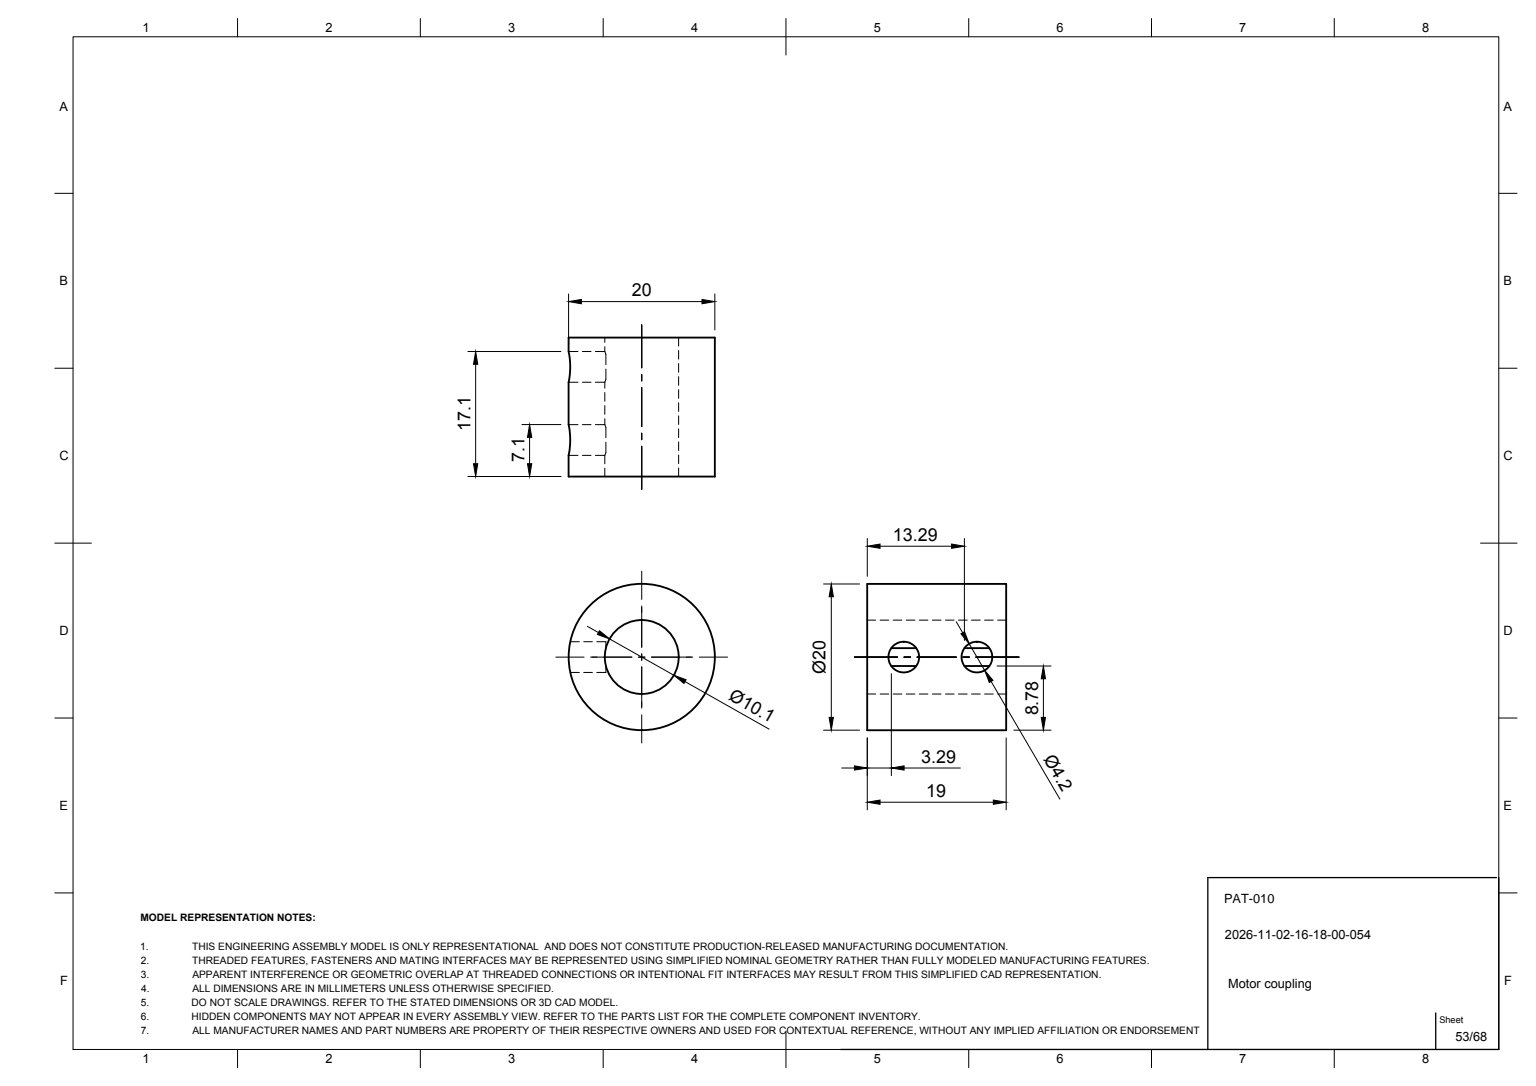
ISO-10303-21;
HEADER;
/* Generated by software containing ST-Developer
 * from STEP Tools, Inc. (www.steptools.com) 
 */

FILE_DESCRIPTION(
/* description */ ('Belt conveyor head drive unit'),
/* implementation_level */ '2;1');

FILE_NAME(
/* name */ 'Motor coupling.step',
/* time_stamp */ '2026-10-28T03:26:19-07:00',
/* author */ (''),
/* organization */ (''),
/* preprocessor_version */ 'ST-DEVELOPER v20.2',
/* originating_system */ 'Autodesk Translation Framework v15.17.0.0',
/* authorisation */ '');

FILE_SCHEMA (('AUTOMOTIVE_DESIGN { 1 0 10303 214 3 1 1 }'));
ENDSEC;

DATA;
#10=MECHANICAL_DESIGN_GEOMETRIC_PRESENTATION_REPRESENTATION('',(#914),#27069);
#577=B_SPLINE_CURVE_WITH_KNOTS('',3,(#24565,#24566,#24567,#24568,#24569,
#24570,#24571,#24572,#24573,#24574),.UNSPECIFIED.,.F.,.F.,(4,2,2,2,4),(0.83629428206811,
0.881958251377254,0.962083854030852,1.04220945668445,1.08787342599359),
 .UNSPECIFIED.);
#578=B_SPLINE_CURVE_WITH_KNOTS('',3,(#24580,#24581,#24582,#24583,#24584,
#24585,#24586,#24587,#24588,#24589,#24590,#24591,#24592,#24593,#24594,#24595,
#24596,#24597),.UNSPECIFIED.,.F.,.F.,(4,2,2,2,2,2,2,2,4),(0.,0.0793616477694785,
0.158723295538957,0.238079516586307,0.317435737633656,0.396791958681006,
0.476148179728355,0.555509827497834,0.634871475267312),.UNSPECIFIED.);
#579=B_SPLINE_CURVE_WITH_KNOTS('',3,(#24598,#24599,#24600,#24601,#24602,
#24603,#24604,#24605,#24606,#24607,#24608,#24609,#24610,#24611,#24612,#24613,
#24614,#24615),.UNSPECIFIED.,.F.,.F.,(4,2,2,2,2,2,2,2,4),(0.634871475267312,
0.714233123036791,0.793594770806269,0.872950991853619,0.952307212900968,
1.03166343394832,1.11101965499567,1.19038130276515,1.26974295053462),
 .UNSPECIFIED.);
#580=B_SPLINE_CURVE_WITH_KNOTS('',3,(#24618,#24619,#24620,#24621,#24622,
#24623,#24624,#24625,#24626,#24627),.UNSPECIFIED.,.F.,.F.,(4,2,2,2,4),(0.194905046047542,
0.240569015356686,0.320694618010284,0.400820220663882,0.446484189973025),
 .UNSPECIFIED.);
#581=B_SPLINE_CURVE_WITH_KNOTS('',3,(#24637,#24638,#24639,#24640,#24641,
#24642,#24643,#24644,#24645,#24646),.UNSPECIFIED.,.F.,.F.,(4,2,2,2,4),(0.83629428206811,
0.881958251377254,0.962083854030852,1.04220945668445,1.08787342599359),
 .UNSPECIFIED.);
#582=B_SPLINE_CURVE_WITH_KNOTS('',3,(#24652,#24653,#24654,#24655,#24656,
#24657,#24658,#24659,#24660,#24661,#24662,#24663,#24664,#24665,#24666,#24667,
#24668,#24669),.UNSPECIFIED.,.F.,.F.,(4,2,2,2,2,2,2,2,4),(0.,0.0793616477694785,
0.158723295538957,0.238079516586307,0.317435737633656,0.396791958681006,
0.476148179728355,0.555509827497834,0.634871475267312),.UNSPECIFIED.);
#583=B_SPLINE_CURVE_WITH_KNOTS('',3,(#24670,#24671,#24672,#24673,#24674,
#24675,#24676,#24677,#24678,#24679,#24680,#24681,#24682,#24683,#24684,#24685,
#24686,#24687),.UNSPECIFIED.,.F.,.F.,(4,2,2,2,2,2,2,2,4),(0.634871475267312,
0.714233123036791,0.793594770806269,0.872950991853619,0.952307212900968,
1.03166343394832,1.11101965499567,1.19038130276515,1.26974295053462),
 .UNSPECIFIED.);
#584=B_SPLINE_CURVE_WITH_KNOTS('',3,(#24690,#24691,#24692,#24693,#24694,
#24695,#24696,#24697,#24698,#24699),.UNSPECIFIED.,.F.,.F.,(4,2,2,2,4),(0.194905046047542,
0.240569015356686,0.320694618010284,0.400820220663882,0.446484189973025),
 .UNSPECIFIED.);
#760=SHAPE_REPRESENTATION_RELATIONSHIP('SRR','None',#27408,#829);
#829=ADVANCED_BREP_SHAPE_REPRESENTATION('',(#995),#27050);
#914=STYLED_ITEM('',(#27783),#995);
#995=MANIFOLD_SOLID_BREP('Body1',#13783);
#1216=FACE_BOUND('',#3192,.T.);
#1217=FACE_BOUND('',#3193,.T.);
#1218=FACE_BOUND('',#3195,.T.);
#1219=FACE_BOUND('',#3196,.T.);
#1220=FACE_BOUND('',#3198,.T.);
#1221=FACE_BOUND('',#3200,.T.);
#1560=PLANE('',#15709);
#1561=PLANE('',#15714);
#1562=PLANE('',#15715);
#1563=PLANE('',#15720);
#1564=PLANE('',#15727);
#1565=PLANE('',#15728);
#2181=FACE_OUTER_BOUND('',#3185,.T.);
#2182=FACE_OUTER_BOUND('',#3186,.T.);
#2183=FACE_OUTER_BOUND('',#3187,.T.);
#2184=FACE_OUTER_BOUND('',#3188,.T.);
#2185=FACE_OUTER_BOUND('',#3189,.T.);
#2186=FACE_OUTER_BOUND('',#3190,.T.);
#2187=FACE_OUTER_BOUND('',#3191,.T.);
#2188=FACE_OUTER_BOUND('',#3194,.T.);
#2189=FACE_OUTER_BOUND('',#3197,.T.);
#2190=FACE_OUTER_BOUND('',#3199,.T.);
#3185=EDGE_LOOP('',(#11250,#11251));
#3186=EDGE_LOOP('',(#11252,#11253,#11254,#11255,#11256,#11257,#11258,#11259,
#11260));
#3187=EDGE_LOOP('',(#11261,#11262,#11263));
#3188=EDGE_LOOP('',(#11264,#11265));
#3189=EDGE_LOOP('',(#11266,#11267,#11268,#11269,#11270,#11271,#11272,#11273,
#11274));
#3190=EDGE_LOOP('',(#11275,#11276,#11277));
#3191=EDGE_LOOP('',(#11278,#11279,#11280,#11281));
#3192=EDGE_LOOP('',(#11282,#11283,#11284,#11285));
#3193=EDGE_LOOP('',(#11286,#11287,#11288,#11289));
#3194=EDGE_LOOP('',(#11290,#11291,#11292,#11293));
#3195=EDGE_LOOP('',(#11294,#11295));
#3196=EDGE_LOOP('',(#11296,#11297));
#3197=EDGE_LOOP('',(#11298));
#3198=EDGE_LOOP('',(#11299));
#3199=EDGE_LOOP('',(#11300));
#3200=EDGE_LOOP('',(#11301));
#4059=LINE('',#24561,#4851);
#4060=LINE('',#24578,#4852);
#4061=LINE('',#24629,#4853);
#4062=LINE('',#24633,#4854);
#4063=LINE('',#24650,#4855);
#4064=LINE('',#24701,#4856);
#4065=LINE('',#24706,#4857);
#4066=LINE('',#24712,#4858);
#4851=VECTOR('',#19291,1.);
#4852=VECTOR('',#19298,0.21);
#4853=VECTOR('',#19303,1.);
#4854=VECTOR('',#19306,1.);
#4855=VECTOR('',#19313,0.21);
#4856=VECTOR('',#19318,1.);
#4857=VECTOR('',#19323,0.505);
#4858=VECTOR('',#19330,1.);
#5611=CIRCLE('',#15710,0.21);
#5612=CIRCLE('',#15712,0.21);
#5613=CIRCLE('',#15713,0.21);
#5614=CIRCLE('',#15716,0.21);
#5615=CIRCLE('',#15718,0.21);
#5616=CIRCLE('',#15719,0.21);
#5617=CIRCLE('',#15722,0.505);
#5618=CIRCLE('',#15723,0.505);
#5619=CIRCLE('',#15725,1.);
#5620=CIRCLE('',#15726,1.);
#6737=VERTEX_POINT('',#24559);
#6738=VERTEX_POINT('',#24560);
#6739=VERTEX_POINT('',#24564);
#6740=VERTEX_POINT('',#24575);
#6741=VERTEX_POINT('',#24577);
#6742=VERTEX_POINT('',#24579);
#6743=VERTEX_POINT('',#24616);
#6744=VERTEX_POINT('',#24631);
#6745=VERTEX_POINT('',#24632);
#6746=VERTEX_POINT('',#24636);
#6747=VERTEX_POINT('',#24647);
#6748=VERTEX_POINT('',#24649);
#6749=VERTEX_POINT('',#24651);
#6750=VERTEX_POINT('',#24688);
#6751=VERTEX_POINT('',#24703);
#6752=VERTEX_POINT('',#24705);
#6753=VERTEX_POINT('',#24709);
#6754=VERTEX_POINT('',#24711);
#8317=EDGE_CURVE('',#6737,#6738,#4059,.T.);
#8318=EDGE_CURVE('',#6737,#6738,#5611,.T.);
#8319=EDGE_CURVE('',#6739,#6737,#577,.T.);
#8320=EDGE_CURVE('',#6740,#6739,#5612,.T.);
#8321=EDGE_CURVE('',#6740,#6741,#4060,.T.);
#8322=EDGE_CURVE('',#6742,#6741,#578,.T.);
#8323=EDGE_CURVE('',#6741,#6742,#579,.T.);
#8324=EDGE_CURVE('',#6743,#6740,#5613,.T.);
#8325=EDGE_CURVE('',#6738,#6743,#580,.T.);
#8326=EDGE_CURVE('',#6743,#6739,#4061,.T.);
#8327=EDGE_CURVE('',#6744,#6745,#4062,.T.);
#8328=EDGE_CURVE('',#6744,#6745,#5614,.T.);
#8329=EDGE_CURVE('',#6746,#6744,#581,.T.);
#8330=EDGE_CURVE('',#6747,#6746,#5615,.T.);
#8331=EDGE_CURVE('',#6747,#6748,#4063,.T.);
#8332=EDGE_CURVE('',#6749,#6748,#582,.T.);
#8333=EDGE_CURVE('',#6748,#6749,#583,.T.);
#8334=EDGE_CURVE('',#6750,#6747,#5616,.T.);
#8335=EDGE_CURVE('',#6745,#6750,#584,.T.);
#8336=EDGE_CURVE('',#6750,#6746,#4064,.T.);
#8337=EDGE_CURVE('',#6751,#6751,#5617,.T.);
#8338=EDGE_CURVE('',#6751,#6752,#4065,.T.);
#8339=EDGE_CURVE('',#6752,#6752,#5618,.T.);
#8340=EDGE_CURVE('',#6753,#6753,#5619,.T.);
#8341=EDGE_CURVE('',#6753,#6754,#4066,.T.);
#8342=EDGE_CURVE('',#6754,#6754,#5620,.T.);
#11250=ORIENTED_EDGE('',*,*,#8317,.F.);
#11251=ORIENTED_EDGE('',*,*,#8318,.T.);
#11252=ORIENTED_EDGE('',*,*,#8319,.F.);
#11253=ORIENTED_EDGE('',*,*,#8320,.F.);
#11254=ORIENTED_EDGE('',*,*,#8321,.T.);
#11255=ORIENTED_EDGE('',*,*,#8322,.F.);
#11256=ORIENTED_EDGE('',*,*,#8323,.F.);
#11257=ORIENTED_EDGE('',*,*,#8321,.F.);
#11258=ORIENTED_EDGE('',*,*,#8324,.F.);
#11259=ORIENTED_EDGE('',*,*,#8325,.F.);
#11260=ORIENTED_EDGE('',*,*,#8318,.F.);
#11261=ORIENTED_EDGE('',*,*,#8326,.F.);
#11262=ORIENTED_EDGE('',*,*,#8324,.T.);
#11263=ORIENTED_EDGE('',*,*,#8320,.T.);
#11264=ORIENTED_EDGE('',*,*,#8327,.F.);
#11265=ORIENTED_EDGE('',*,*,#8328,.T.);
#11266=ORIENTED_EDGE('',*,*,#8329,.F.);
#11267=ORIENTED_EDGE('',*,*,#8330,.F.);
#11268=ORIENTED_EDGE('',*,*,#8331,.T.);
#11269=ORIENTED_EDGE('',*,*,#8332,.F.);
#11270=ORIENTED_EDGE('',*,*,#8333,.F.);
#11271=ORIENTED_EDGE('',*,*,#8331,.F.);
#11272=ORIENTED_EDGE('',*,*,#8334,.F.);
#11273=ORIENTED_EDGE('',*,*,#8335,.F.);
#11274=ORIENTED_EDGE('',*,*,#8328,.F.);
#11275=ORIENTED_EDGE('',*,*,#8336,.F.);
#11276=ORIENTED_EDGE('',*,*,#8334,.T.);
#11277=ORIENTED_EDGE('',*,*,#8330,.T.);
#11278=ORIENTED_EDGE('',*,*,#8337,.F.);
#11279=ORIENTED_EDGE('',*,*,#8338,.T.);
#11280=ORIENTED_EDGE('',*,*,#8339,.T.);
#11281=ORIENTED_EDGE('',*,*,#8338,.F.);
#11282=ORIENTED_EDGE('',*,*,#8325,.T.);
#11283=ORIENTED_EDGE('',*,*,#8326,.T.);
#11284=ORIENTED_EDGE('',*,*,#8319,.T.);
#11285=ORIENTED_EDGE('',*,*,#8317,.T.);
#11286=ORIENTED_EDGE('',*,*,#8335,.T.);
#11287=ORIENTED_EDGE('',*,*,#8336,.T.);
#11288=ORIENTED_EDGE('',*,*,#8329,.T.);
#11289=ORIENTED_EDGE('',*,*,#8327,.T.);
#11290=ORIENTED_EDGE('',*,*,#8340,.F.);
#11291=ORIENTED_EDGE('',*,*,#8341,.T.);
#11292=ORIENTED_EDGE('',*,*,#8342,.T.);
#11293=ORIENTED_EDGE('',*,*,#8341,.F.);
#11294=ORIENTED_EDGE('',*,*,#8322,.T.);
#11295=ORIENTED_EDGE('',*,*,#8323,.T.);
#11296=ORIENTED_EDGE('',*,*,#8332,.T.);
#11297=ORIENTED_EDGE('',*,*,#8333,.T.);
#11298=ORIENTED_EDGE('',*,*,#8340,.T.);
#11299=ORIENTED_EDGE('',*,*,#8337,.T.);
#11300=ORIENTED_EDGE('',*,*,#8342,.F.);
#11301=ORIENTED_EDGE('',*,*,#8339,.F.);
#12739=CYLINDRICAL_SURFACE('',#15711,0.21);
#12740=CYLINDRICAL_SURFACE('',#15717,0.21);
#12741=CYLINDRICAL_SURFACE('',#15721,0.505);
#12742=CYLINDRICAL_SURFACE('',#15724,1.);
#13460=ADVANCED_FACE('',(#2181),#1560,.T.);
#13461=ADVANCED_FACE('',(#2182),#12739,.F.);
#13462=ADVANCED_FACE('',(#2183),#1561,.T.);
#13463=ADVANCED_FACE('',(#2184),#1562,.T.);
#13464=ADVANCED_FACE('',(#2185),#12740,.F.);
#13465=ADVANCED_FACE('',(#2186),#1563,.T.);
#13466=ADVANCED_FACE('',(#2187,#1216,#1217),#12741,.F.);
#13467=ADVANCED_FACE('',(#2188,#1218,#1219),#12742,.T.);
#13468=ADVANCED_FACE('',(#2189,#1220),#1564,.T.);
#13469=ADVANCED_FACE('',(#2190,#1221),#1565,.F.);
#13783=CLOSED_SHELL('',(#13460,#13461,#13462,#13463,#13464,#13465,#13466,
#13467,#13468,#13469));
#15708=AXIS2_PLACEMENT_3D('',#24557,#19287,#19288);
#15709=AXIS2_PLACEMENT_3D('',#24558,#19289,#19290);
#15710=AXIS2_PLACEMENT_3D('',#24562,#19292,#19293);
#15711=AXIS2_PLACEMENT_3D('',#24563,#19294,#19295);
#15712=AXIS2_PLACEMENT_3D('',#24576,#19296,#19297);
#15713=AXIS2_PLACEMENT_3D('',#24617,#19299,#19300);
#15714=AXIS2_PLACEMENT_3D('',#24628,#19301,#19302);
#15715=AXIS2_PLACEMENT_3D('',#24630,#19304,#19305);
#15716=AXIS2_PLACEMENT_3D('',#24634,#19307,#19308);
#15717=AXIS2_PLACEMENT_3D('',#24635,#19309,#19310);
#15718=AXIS2_PLACEMENT_3D('',#24648,#19311,#19312);
#15719=AXIS2_PLACEMENT_3D('',#24689,#19314,#19315);
#15720=AXIS2_PLACEMENT_3D('',#24700,#19316,#19317);
#15721=AXIS2_PLACEMENT_3D('',#24702,#19319,#19320);
#15722=AXIS2_PLACEMENT_3D('',#24704,#19321,#19322);
#15723=AXIS2_PLACEMENT_3D('',#24707,#19324,#19325);
#15724=AXIS2_PLACEMENT_3D('',#24708,#19326,#19327);
#15725=AXIS2_PLACEMENT_3D('',#24710,#19328,#19329);
#15726=AXIS2_PLACEMENT_3D('',#24713,#19331,#19332);
#15727=AXIS2_PLACEMENT_3D('',#24714,#19333,#19334);
#15728=AXIS2_PLACEMENT_3D('',#24715,#19335,#19336);
#19287=DIRECTION('axis',(0.,0.,1.));
#19288=DIRECTION('refdir',(1.,0.,0.));
#19289=DIRECTION('center_axis',(0.,0.,1.));
#19290=DIRECTION('ref_axis',(1.,0.,0.));
#19291=DIRECTION('',(0.,1.,0.));
#19292=DIRECTION('center_axis',(0.,0.,1.));
#19293=DIRECTION('ref_axis',(1.,0.,0.));
#19294=DIRECTION('center_axis',(0.,0.,1.));
#19295=DIRECTION('ref_axis',(1.,0.,0.));
#19296=DIRECTION('center_axis',(0.,0.,1.));
#19297=DIRECTION('ref_axis',(1.,0.,0.));
#19298=DIRECTION('',(0.,0.,1.));
#19299=DIRECTION('center_axis',(0.,0.,1.));
#19300=DIRECTION('ref_axis',(1.,0.,0.));
#19301=DIRECTION('center_axis',(0.,0.,1.));
#19302=DIRECTION('ref_axis',(1.,0.,0.));
#19303=DIRECTION('',(0.,-1.,0.));
#19304=DIRECTION('center_axis',(0.,0.,1.));
#19305=DIRECTION('ref_axis',(1.,0.,0.));
#19306=DIRECTION('',(0.,1.,0.));
#19307=DIRECTION('center_axis',(0.,0.,1.));
#19308=DIRECTION('ref_axis',(1.,0.,0.));
#19309=DIRECTION('center_axis',(0.,0.,1.));
#19310=DIRECTION('ref_axis',(1.,0.,0.));
#19311=DIRECTION('center_axis',(0.,0.,1.));
#19312=DIRECTION('ref_axis',(1.,0.,0.));
#19313=DIRECTION('',(0.,0.,1.));
#19314=DIRECTION('center_axis',(0.,0.,1.));
#19315=DIRECTION('ref_axis',(1.,0.,0.));
#19316=DIRECTION('center_axis',(0.,0.,1.));
#19317=DIRECTION('ref_axis',(1.,0.,0.));
#19318=DIRECTION('',(0.,-1.,0.));
#19319=DIRECTION('center_axis',(0.,1.,0.));
#19320=DIRECTION('ref_axis',(1.,0.,0.));
#19321=DIRECTION('center_axis',(0.,-1.,0.));
#19322=DIRECTION('ref_axis',(1.,0.,0.));
#19323=DIRECTION('',(0.,-1.,0.));
#19324=DIRECTION('center_axis',(0.,-1.,0.));
#19325=DIRECTION('ref_axis',(1.,0.,0.));
#19326=DIRECTION('center_axis',(0.,1.,0.));
#19327=DIRECTION('ref_axis',(1.,0.,0.));
#19328=DIRECTION('center_axis',(0.,1.,0.));
#19329=DIRECTION('ref_axis',(1.,0.,0.));
#19330=DIRECTION('',(0.,-1.,0.));
#19331=DIRECTION('center_axis',(0.,1.,0.));
#19332=DIRECTION('ref_axis',(1.,0.,0.));
#19333=DIRECTION('center_axis',(0.,1.,0.));
#19334=DIRECTION('ref_axis',(1.,0.,0.));
#19335=DIRECTION('center_axis',(0.,1.,0.));
#19336=DIRECTION('ref_axis',(1.,0.,0.));
#24557=CARTESIAN_POINT('',(0.,0.,0.));
#24558=CARTESIAN_POINT('Origin',(0.,3.5,7.49));
#24559=CARTESIAN_POINT('',(0.122167917228702,3.32919309147461,7.49));
#24560=CARTESIAN_POINT('',(0.122167917228702,3.67080690852539,7.49));
#24561=CARTESIAN_POINT('',(0.122167917228702,2.1,7.49));
#24562=CARTESIAN_POINT('Origin',(0.,3.5,7.49));
#24563=CARTESIAN_POINT('Origin',(0.,3.5,7.49));
#24564=CARTESIAN_POINT('',(-0.122167917228702,3.32919309147461,7.49));
#24565=CARTESIAN_POINT('Ctrl Pts',(-0.122167917228702,3.32919309147461,
7.49));
#24566=CARTESIAN_POINT('Ctrl Pts',(-0.109498349122107,3.3201313107707,7.49315880560769));
#24567=CARTESIAN_POINT('Ctrl Pts',(-0.0955290239036627,3.31230742432584,
7.49610638003428));
#24568=CARTESIAN_POINT('Ctrl Pts',(-0.0549836006623198,3.29540341787373,
7.50267917175998));
#24569=CARTESIAN_POINT('Ctrl Pts',(-0.0267085342178658,3.29,7.505));
#24570=CARTESIAN_POINT('Ctrl Pts',(0.0267085342178659,3.29,7.505));
#24571=CARTESIAN_POINT('Ctrl Pts',(0.0549836006623198,3.29540341787373,
7.50267917175998));
#24572=CARTESIAN_POINT('Ctrl Pts',(0.0955290239036627,3.31230742432584,
7.49610638003428));
#24573=CARTESIAN_POINT('Ctrl Pts',(0.109498349122108,3.3201313107707,7.49315880560769));
#24574=CARTESIAN_POINT('Ctrl Pts',(0.122167917228702,3.32919309147461,7.49));
#24575=CARTESIAN_POINT('',(-0.21,3.5,7.49));
#24576=CARTESIAN_POINT('Origin',(0.,3.5,7.49));
#24577=CARTESIAN_POINT('',(-0.21,3.5,7.97770138590472));
#24578=CARTESIAN_POINT('',(-0.21,3.5,7.49));
#24579=CARTESIAN_POINT('',(0.21,3.5,7.97770138590472));
#24580=CARTESIAN_POINT('Ctrl Pts',(0.21,3.5,7.97770138590472));
#24581=CARTESIAN_POINT('Ctrl Pts',(0.21,3.47354611741017,7.97770138590472));
#24582=CARTESIAN_POINT('Ctrl Pts',(0.204697017125528,3.44538474169131,7.97888646613217));
#24583=CARTESIAN_POINT('Ctrl Pts',(0.183241751515529,3.39366957869826,7.98312869991148));
#24584=CARTESIAN_POINT('Ctrl Pts',(0.167093586802906,3.37010873870456,7.98612044796649));
#24585=CARTESIAN_POINT('Ctrl Pts',(0.129892533236543,3.33290768513819,7.99170645156379));
#24586=CARTESIAN_POINT('Ctrl Pts',(0.106331154992714,3.31675852489431,7.99466914446598));
#24587=CARTESIAN_POINT('Ctrl Pts',(0.0546141143983531,3.29530253627557,
7.99884449237241));
#24588=CARTESIAN_POINT('Ctrl Pts',(0.0264520736824499,3.29,8.));
#24589=CARTESIAN_POINT('Ctrl Pts',(-0.0264520736824498,3.29,8.));
#24590=CARTESIAN_POINT('Ctrl Pts',(-0.054614114398353,3.29530253627557,
7.99884449237241));
#24591=CARTESIAN_POINT('Ctrl Pts',(-0.106331154992714,3.31675852489431,
7.99466914446598));
#24592=CARTESIAN_POINT('Ctrl Pts',(-0.129892533236543,3.33290768513819,
7.99170645156379));
#24593=CARTESIAN_POINT('Ctrl Pts',(-0.167093586802906,3.37010873870456,
7.98612044796649));
#24594=CARTESIAN_POINT('Ctrl Pts',(-0.183241751515529,3.39366957869826,
7.98312869991148));
#24595=CARTESIAN_POINT('Ctrl Pts',(-0.204697017125528,3.44538474169131,
7.97888646613217));
#24596=CARTESIAN_POINT('Ctrl Pts',(-0.21,3.47354611741017,7.97770138590472));
#24597=CARTESIAN_POINT('Ctrl Pts',(-0.21,3.5,7.97770138590472));
#24598=CARTESIAN_POINT('Ctrl Pts',(-0.21,3.5,7.97770138590472));
#24599=CARTESIAN_POINT('Ctrl Pts',(-0.21,3.52645388258983,7.97770138590472));
#24600=CARTESIAN_POINT('Ctrl Pts',(-0.204697017125528,3.55461525830869,
7.97888646613217));
#24601=CARTESIAN_POINT('Ctrl Pts',(-0.183241751515529,3.60633042130174,
7.98312869991148));
#24602=CARTESIAN_POINT('Ctrl Pts',(-0.167093586802906,3.62989126129544,
7.98612044796649));
#24603=CARTESIAN_POINT('Ctrl Pts',(-0.129892533236543,3.66709231486181,
7.99170645156379));
#24604=CARTESIAN_POINT('Ctrl Pts',(-0.106331154992714,3.68324147510569,
7.99466914446598));
#24605=CARTESIAN_POINT('Ctrl Pts',(-0.0546141143983532,3.70469746372443,
7.99884449237241));
#24606=CARTESIAN_POINT('Ctrl Pts',(-0.0264520736824499,3.71,8.));
#24607=CARTESIAN_POINT('Ctrl Pts',(0.0264520736824498,3.71,8.));
#24608=CARTESIAN_POINT('Ctrl Pts',(0.0546141143983531,3.70469746372443,
7.99884449237241));
#24609=CARTESIAN_POINT('Ctrl Pts',(0.106331154992714,3.68324147510569,7.99466914446598));
#24610=CARTESIAN_POINT('Ctrl Pts',(0.129892533236543,3.66709231486181,7.99170645156379));
#24611=CARTESIAN_POINT('Ctrl Pts',(0.167093586802906,3.62989126129544,7.98612044796649));
#24612=CARTESIAN_POINT('Ctrl Pts',(0.183241751515529,3.60633042130174,7.98312869991148));
#24613=CARTESIAN_POINT('Ctrl Pts',(0.204697017125528,3.55461525830869,7.97888646613217));
#24614=CARTESIAN_POINT('Ctrl Pts',(0.21,3.52645388258983,7.97770138590472));
#24615=CARTESIAN_POINT('Ctrl Pts',(0.21,3.5,7.97770138590472));
#24616=CARTESIAN_POINT('',(-0.122167917228702,3.67080690852539,7.49));
#24617=CARTESIAN_POINT('Origin',(0.,3.5,7.49));
#24618=CARTESIAN_POINT('Ctrl Pts',(0.122167917228702,3.67080690852539,7.49));
#24619=CARTESIAN_POINT('Ctrl Pts',(0.109498349122108,3.6798686892293,7.49315880560769));
#24620=CARTESIAN_POINT('Ctrl Pts',(0.0955290239036627,3.68769257567416,
7.49610638003428));
#24621=CARTESIAN_POINT('Ctrl Pts',(0.0549836006623198,3.70459658212627,
7.50267917175998));
#24622=CARTESIAN_POINT('Ctrl Pts',(0.0267085342178658,3.71,7.505));
#24623=CARTESIAN_POINT('Ctrl Pts',(-0.0267085342178659,3.71,7.505));
#24624=CARTESIAN_POINT('Ctrl Pts',(-0.0549836006623198,3.70459658212627,
7.50267917175998));
#24625=CARTESIAN_POINT('Ctrl Pts',(-0.0955290239036627,3.68769257567416,
7.49610638003428));
#24626=CARTESIAN_POINT('Ctrl Pts',(-0.109498349122107,3.6798686892293,7.49315880560769));
#24627=CARTESIAN_POINT('Ctrl Pts',(-0.122167917228702,3.67080690852539,
7.49));
#24628=CARTESIAN_POINT('Origin',(0.,3.5,7.49));
#24629=CARTESIAN_POINT('',(-0.122167917228702,2.1,7.49));
#24630=CARTESIAN_POINT('Origin',(0.,2.5,7.49));
#24631=CARTESIAN_POINT('',(0.122167917228702,2.32919309147461,7.49));
#24632=CARTESIAN_POINT('',(0.122167917228702,2.67080690852539,7.49));
#24633=CARTESIAN_POINT('',(0.122167917228702,2.1,7.49));
#24634=CARTESIAN_POINT('Origin',(0.,2.5,7.49));
#24635=CARTESIAN_POINT('Origin',(0.,2.5,7.49));
#24636=CARTESIAN_POINT('',(-0.122167917228702,2.32919309147461,7.49));
#24637=CARTESIAN_POINT('Ctrl Pts',(-0.122167917228702,2.32919309147461,
7.49));
#24638=CARTESIAN_POINT('Ctrl Pts',(-0.109498349122107,2.3201313107707,7.49315880560769));
#24639=CARTESIAN_POINT('Ctrl Pts',(-0.0955290239036627,2.31230742432584,
7.49610638003428));
#24640=CARTESIAN_POINT('Ctrl Pts',(-0.0549836006623198,2.29540341787373,
7.50267917175998));
#24641=CARTESIAN_POINT('Ctrl Pts',(-0.0267085342178658,2.29,7.505));
#24642=CARTESIAN_POINT('Ctrl Pts',(0.0267085342178659,2.29,7.505));
#24643=CARTESIAN_POINT('Ctrl Pts',(0.0549836006623198,2.29540341787373,
7.50267917175998));
#24644=CARTESIAN_POINT('Ctrl Pts',(0.0955290239036627,2.31230742432584,
7.49610638003428));
#24645=CARTESIAN_POINT('Ctrl Pts',(0.109498349122107,2.3201313107707,7.49315880560769));
#24646=CARTESIAN_POINT('Ctrl Pts',(0.122167917228702,2.32919309147461,7.49));
#24647=CARTESIAN_POINT('',(-0.21,2.5,7.49));
#24648=CARTESIAN_POINT('Origin',(0.,2.5,7.49));
#24649=CARTESIAN_POINT('',(-0.21,2.5,7.97770138590472));
#24650=CARTESIAN_POINT('',(-0.21,2.5,7.49));
#24651=CARTESIAN_POINT('',(0.21,2.5,7.97770138590472));
#24652=CARTESIAN_POINT('Ctrl Pts',(0.21,2.5,7.97770138590472));
#24653=CARTESIAN_POINT('Ctrl Pts',(0.21,2.47354611741017,7.97770138590472));
#24654=CARTESIAN_POINT('Ctrl Pts',(0.204697017125528,2.44538474169131,7.97888646613217));
#24655=CARTESIAN_POINT('Ctrl Pts',(0.183241751515529,2.39366957869826,7.98312869991148));
#24656=CARTESIAN_POINT('Ctrl Pts',(0.167093586802906,2.37010873870456,7.98612044796649));
#24657=CARTESIAN_POINT('Ctrl Pts',(0.129892533236543,2.33290768513819,7.99170645156379));
#24658=CARTESIAN_POINT('Ctrl Pts',(0.106331154992714,2.31675852489431,7.99466914446598));
#24659=CARTESIAN_POINT('Ctrl Pts',(0.0546141143983531,2.29530253627557,
7.99884449237241));
#24660=CARTESIAN_POINT('Ctrl Pts',(0.0264520736824499,2.29,8.));
#24661=CARTESIAN_POINT('Ctrl Pts',(-0.0264520736824498,2.29,8.));
#24662=CARTESIAN_POINT('Ctrl Pts',(-0.0546141143983532,2.29530253627557,
7.99884449237241));
#24663=CARTESIAN_POINT('Ctrl Pts',(-0.106331154992714,2.31675852489431,
7.99466914446598));
#24664=CARTESIAN_POINT('Ctrl Pts',(-0.129892533236543,2.33290768513819,
7.99170645156379));
#24665=CARTESIAN_POINT('Ctrl Pts',(-0.167093586802906,2.37010873870456,
7.98612044796649));
#24666=CARTESIAN_POINT('Ctrl Pts',(-0.183241751515529,2.39366957869826,
7.98312869991148));
#24667=CARTESIAN_POINT('Ctrl Pts',(-0.204697017125528,2.44538474169131,
7.97888646613217));
#24668=CARTESIAN_POINT('Ctrl Pts',(-0.21,2.47354611741017,7.97770138590472));
#24669=CARTESIAN_POINT('Ctrl Pts',(-0.21,2.5,7.97770138590472));
#24670=CARTESIAN_POINT('Ctrl Pts',(-0.21,2.5,7.97770138590472));
#24671=CARTESIAN_POINT('Ctrl Pts',(-0.21,2.52645388258983,7.97770138590472));
#24672=CARTESIAN_POINT('Ctrl Pts',(-0.204697017125528,2.55461525830869,
7.97888646613217));
#24673=CARTESIAN_POINT('Ctrl Pts',(-0.183241751515529,2.60633042130174,
7.98312869991148));
#24674=CARTESIAN_POINT('Ctrl Pts',(-0.167093586802906,2.62989126129544,
7.98612044796649));
#24675=CARTESIAN_POINT('Ctrl Pts',(-0.129892533236543,2.66709231486181,
7.99170645156379));
#24676=CARTESIAN_POINT('Ctrl Pts',(-0.106331154992714,2.68324147510569,
7.99466914446598));
#24677=CARTESIAN_POINT('Ctrl Pts',(-0.0546141143983532,2.70469746372443,
7.99884449237241));
#24678=CARTESIAN_POINT('Ctrl Pts',(-0.0264520736824499,2.71,8.));
#24679=CARTESIAN_POINT('Ctrl Pts',(0.0264520736824498,2.71,8.));
#24680=CARTESIAN_POINT('Ctrl Pts',(0.0546141143983531,2.70469746372443,
7.99884449237241));
#24681=CARTESIAN_POINT('Ctrl Pts',(0.106331154992714,2.68324147510569,7.99466914446598));
#24682=CARTESIAN_POINT('Ctrl Pts',(0.129892533236543,2.66709231486181,7.99170645156379));
#24683=CARTESIAN_POINT('Ctrl Pts',(0.167093586802906,2.62989126129544,7.98612044796649));
#24684=CARTESIAN_POINT('Ctrl Pts',(0.183241751515529,2.60633042130174,7.98312869991148));
#24685=CARTESIAN_POINT('Ctrl Pts',(0.204697017125528,2.55461525830869,7.97888646613217));
#24686=CARTESIAN_POINT('Ctrl Pts',(0.21,2.52645388258983,7.97770138590472));
#24687=CARTESIAN_POINT('Ctrl Pts',(0.21,2.5,7.97770138590472));
#24688=CARTESIAN_POINT('',(-0.122167917228702,2.67080690852539,7.49));
#24689=CARTESIAN_POINT('Origin',(0.,2.5,7.49));
#24690=CARTESIAN_POINT('Ctrl Pts',(0.122167917228702,2.67080690852539,7.49));
#24691=CARTESIAN_POINT('Ctrl Pts',(0.109498349122107,2.6798686892293,7.49315880560769));
#24692=CARTESIAN_POINT('Ctrl Pts',(0.0955290239036627,2.68769257567416,
7.49610638003428));
#24693=CARTESIAN_POINT('Ctrl Pts',(0.0549836006623198,2.70459658212627,
7.50267917175998));
#24694=CARTESIAN_POINT('Ctrl Pts',(0.0267085342178658,2.71,7.505));
#24695=CARTESIAN_POINT('Ctrl Pts',(-0.0267085342178659,2.71,7.505));
#24696=CARTESIAN_POINT('Ctrl Pts',(-0.0549836006623198,2.70459658212627,
7.50267917175998));
#24697=CARTESIAN_POINT('Ctrl Pts',(-0.0955290239036626,2.68769257567416,
7.49610638003428));
#24698=CARTESIAN_POINT('Ctrl Pts',(-0.109498349122107,2.6798686892293,7.49315880560769));
#24699=CARTESIAN_POINT('Ctrl Pts',(-0.122167917228702,2.67080690852539,
7.49));
#24700=CARTESIAN_POINT('Origin',(0.,2.5,7.49));
#24701=CARTESIAN_POINT('',(-0.122167917228702,2.1,7.49));
#24702=CARTESIAN_POINT('Origin',(0.,2.1,7.));
#24703=CARTESIAN_POINT('',(-0.505,4.,7.));
#24704=CARTESIAN_POINT('Origin',(0.,4.,7.));
#24705=CARTESIAN_POINT('',(-0.505,2.1,7.));
#24706=CARTESIAN_POINT('',(-0.505,2.1,7.));
#24707=CARTESIAN_POINT('Origin',(0.,2.1,7.));
#24708=CARTESIAN_POINT('Origin',(0.,2.1,7.));
#24709=CARTESIAN_POINT('',(-1.,4.,7.));
#24710=CARTESIAN_POINT('Origin',(0.,4.,7.));
#24711=CARTESIAN_POINT('',(-1.,2.1,7.));
#24712=CARTESIAN_POINT('',(-1.,2.1,7.));
#24713=CARTESIAN_POINT('Origin',(0.,2.1,7.));
#24714=CARTESIAN_POINT('Origin',(0.,4.,7.));
#24715=CARTESIAN_POINT('Origin',(0.,2.1,7.));
#26973=UNCERTAINTY_MEASURE_WITH_UNIT(LENGTH_MEASURE(0.001),#27070,
'DISTANCE_ACCURACY_VALUE',
'Maximum model space distance between geometric entities at asserted c
onnectivities');
#26992=UNCERTAINTY_MEASURE_WITH_UNIT(LENGTH_MEASURE(0.001),#27070,
'DISTANCE_ACCURACY_VALUE',
'Maximum model space distance between geometric entities at asserted c
onnectivities');
#27050=(
GEOMETRIC_REPRESENTATION_CONTEXT(3)
GLOBAL_UNCERTAINTY_ASSIGNED_CONTEXT((#26973))
GLOBAL_UNIT_ASSIGNED_CONTEXT((#27070,#27072,#27073))
REPRESENTATION_CONTEXT('','3D')
);
#27069=(
GEOMETRIC_REPRESENTATION_CONTEXT(3)
GLOBAL_UNCERTAINTY_ASSIGNED_CONTEXT((#26992))
GLOBAL_UNIT_ASSIGNED_CONTEXT((#27070,#27072,#27073))
REPRESENTATION_CONTEXT('','3D')
);
#27070=(
LENGTH_UNIT()
NAMED_UNIT(*)
SI_UNIT(.CENTI.,.METRE.)
);
#27072=(
NAMED_UNIT(*)
PLANE_ANGLE_UNIT()
SI_UNIT($,.RADIAN.)
);
#27073=(
NAMED_UNIT(*)
SI_UNIT($,.STERADIAN.)
SOLID_ANGLE_UNIT()
);
#27131=SHAPE_DEFINITION_REPRESENTATION(#27219,#27408);
#27219=PRODUCT_DEFINITION_SHAPE('',$,#27485);
#27408=SHAPE_REPRESENTATION('',(#15708),#27050);
#27427=PRODUCT_DEFINITION_CONTEXT('part definition',#27657,'design');
#27485=PRODUCT_DEFINITION('Motor coupling','Motor coupling',#27561,#27427);
#27561=PRODUCT_DEFINITION_FORMATION('',$,#27716);
#27657=APPLICATION_CONTEXT(
'Core Data for Automotive Mechanical Design Process');
#27658=PRODUCT_CONTEXT('part definition',#27657,'mechanical');
#27716=PRODUCT('Motor coupling','Motor coupling','Motor coupling',(#27658));
#27777=COLOUR_RGB('Light Blue',0.38,0.62,0.78);
#27778=FILL_AREA_STYLE_COLOUR('',#27777);
#27779=FILL_AREA_STYLE('',(#27778));
#27780=SURFACE_STYLE_FILL_AREA(#27779);
#27781=SURFACE_SIDE_STYLE('',(#27780));
#27782=SURFACE_STYLE_USAGE(.BOTH.,#27781);
#27783=PRESENTATION_STYLE_ASSIGNMENT((#27782));
ENDSEC;
END-ISO-10303-21;
